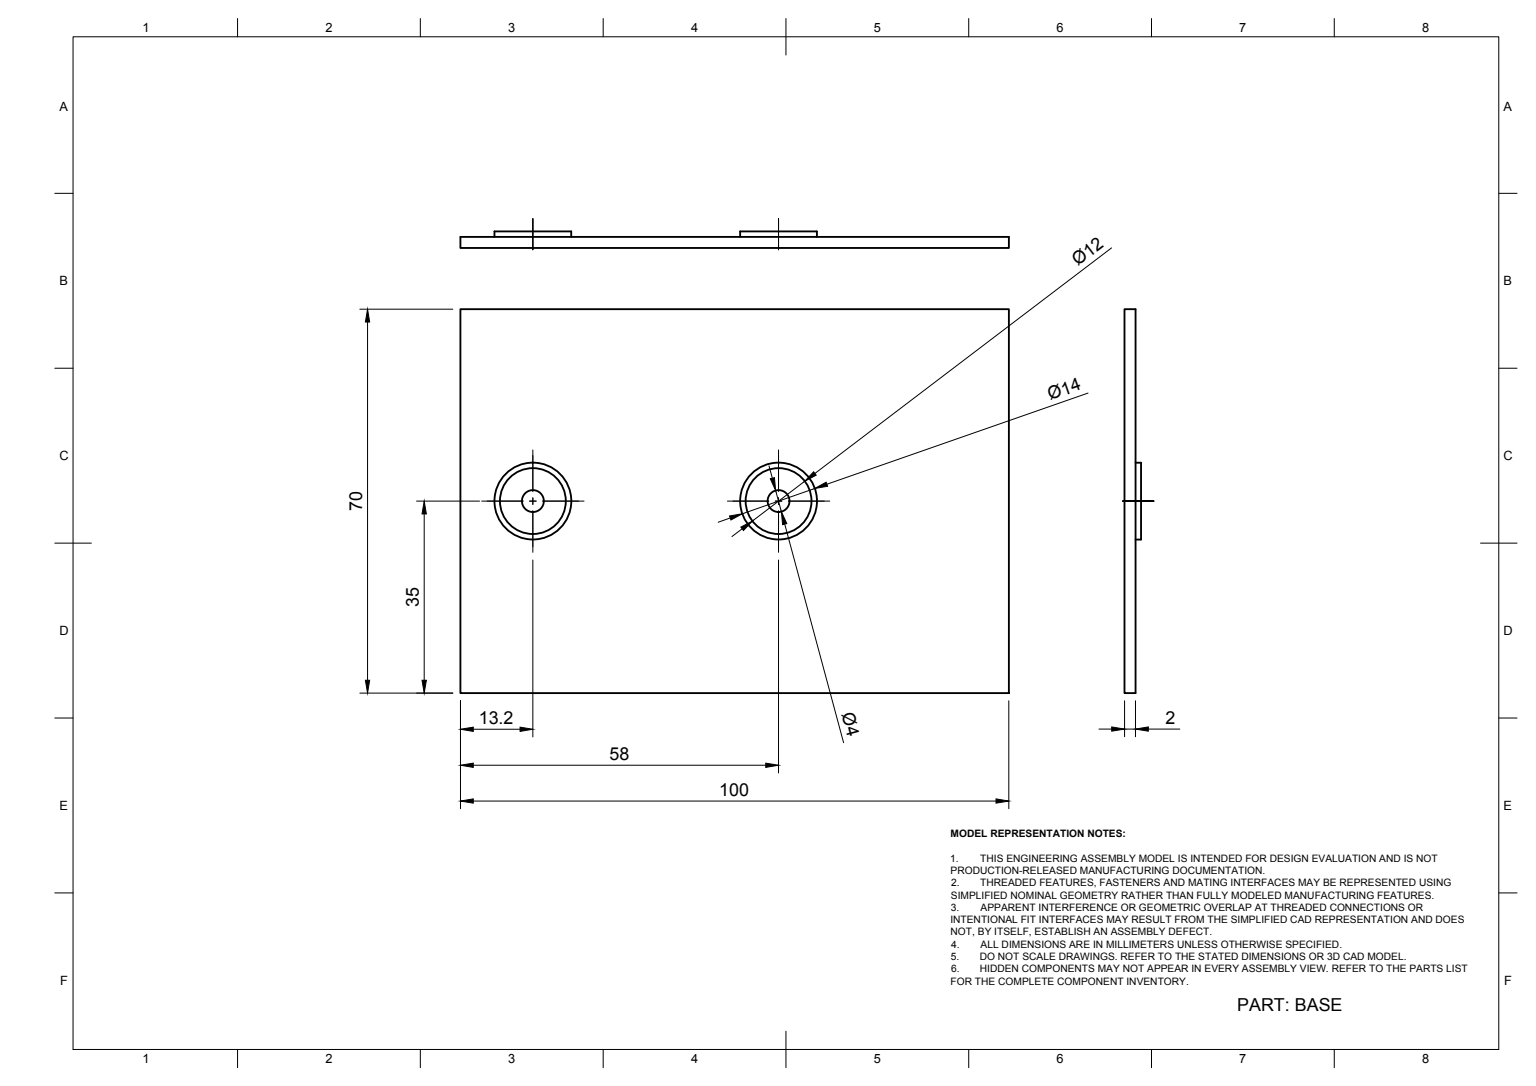
ISO-10303-21;
HEADER;
/* Generated by software containing ST-Developer
 * from STEP Tools, Inc. (www.steptools.com) 
 */

FILE_DESCRIPTION(
/* description */ (''),
/* implementation_level */ '2;1');

FILE_NAME(
/* name */ 'Base.step',
/* time_stamp */ '2026-10-04T15:18:51-07:00',
/* author */ (''),
/* organization */ (''),
/* preprocessor_version */ 'ST-DEVELOPER v20.2',
/* originating_system */ 'Autodesk Translation Framework v15.15.0.0',
/* authorisation */ '');

FILE_SCHEMA (('AUTOMOTIVE_DESIGN { 1 0 10303 214 3 1 1 }'));
ENDSEC;

DATA;
#10=MECHANICAL_DESIGN_GEOMETRIC_PRESENTATION_REPRESENTATION('',(#73),#9891);
#54=SHAPE_REPRESENTATION_RELATIONSHIP('SRR','None',#9925,#62);
#62=ADVANCED_BREP_SHAPE_REPRESENTATION('',(#87),#9885);
#73=STYLED_ITEM('',(#9974),#87);
#87=MANIFOLD_SOLID_BREP('Body1',#5621);
#115=FACE_BOUND('',#834,.T.);
#116=FACE_BOUND('',#836,.T.);
#117=FACE_BOUND('',#837,.T.);
#118=FACE_BOUND('',#841,.T.);
#119=FACE_BOUND('',#843,.T.);
#120=FACE_BOUND('',#849,.T.);
#121=FACE_BOUND('',#850,.T.);
#122=FACE_BOUND('',#852,.T.);
#186=PLANE('',#5903);
#187=PLANE('',#5904);
#188=PLANE('',#5911);
#189=PLANE('',#5912);
#190=PLANE('',#5913);
#191=PLANE('',#5914);
#192=PLANE('',#5915);
#193=PLANE('',#5916);
#194=PLANE('',#5917);
#195=PLANE('',#5918);
#480=FACE_OUTER_BOUND('',#829,.T.);
#481=FACE_OUTER_BOUND('',#830,.T.);
#482=FACE_OUTER_BOUND('',#831,.T.);
#483=FACE_OUTER_BOUND('',#832,.T.);
#484=FACE_OUTER_BOUND('',#833,.T.);
#485=FACE_OUTER_BOUND('',#835,.T.);
#486=FACE_OUTER_BOUND('',#838,.T.);
#487=FACE_OUTER_BOUND('',#839,.T.);
#488=FACE_OUTER_BOUND('',#840,.T.);
#489=FACE_OUTER_BOUND('',#842,.T.);
#490=FACE_OUTER_BOUND('',#844,.T.);
#491=FACE_OUTER_BOUND('',#845,.T.);
#492=FACE_OUTER_BOUND('',#846,.T.);
#493=FACE_OUTER_BOUND('',#847,.T.);
#494=FACE_OUTER_BOUND('',#848,.T.);
#495=FACE_OUTER_BOUND('',#851,.T.);
#829=EDGE_LOOP('',(#3906,#3907,#3908,#3909));
#830=EDGE_LOOP('',(#3910,#3911,#3912,#3913));
#831=EDGE_LOOP('',(#3914,#3915,#3916,#3917));
#832=EDGE_LOOP('',(#3918,#3919,#3920,#3921));
#833=EDGE_LOOP('',(#3922));
#834=EDGE_LOOP('',(#3923));
#835=EDGE_LOOP('',(#3924,#3925,#3926,#3927));
#836=EDGE_LOOP('',(#3928));
#837=EDGE_LOOP('',(#3929));
#838=EDGE_LOOP('',(#3930,#3931,#3932,#3933));
#839=EDGE_LOOP('',(#3934,#3935,#3936,#3937));
#840=EDGE_LOOP('',(#3938));
#841=EDGE_LOOP('',(#3939));
#842=EDGE_LOOP('',(#3940));
#843=EDGE_LOOP('',(#3941));
#844=EDGE_LOOP('',(#3942,#3943,#3944,#3945));
#845=EDGE_LOOP('',(#3946,#3947,#3948,#3949));
#846=EDGE_LOOP('',(#3950,#3951,#3952,#3953));
#847=EDGE_LOOP('',(#3954,#3955,#3956,#3957));
#848=EDGE_LOOP('',(#3958,#3959,#3960,#3961));
#849=EDGE_LOOP('',(#3962));
#850=EDGE_LOOP('',(#3963));
#851=EDGE_LOOP('',(#3964));
#852=EDGE_LOOP('',(#3965));
#1163=LINE('',#8464,#1627);
#1164=LINE('',#8470,#1628);
#1165=LINE('',#8476,#1629);
#1166=LINE('',#8482,#1630);
#1167=LINE('',#8488,#1631);
#1168=LINE('',#8490,#1632);
#1169=LINE('',#8492,#1633);
#1170=LINE('',#8493,#1634);
#1171=LINE('',#8500,#1635);
#1172=LINE('',#8505,#1636);
#1173=LINE('',#8510,#1637);
#1174=LINE('',#8512,#1638);
#1175=LINE('',#8513,#1639);
#1176=LINE('',#8516,#1640);
#1177=LINE('',#8517,#1641);
#1178=LINE('',#8520,#1642);
#1179=LINE('',#8521,#1643);
#1180=LINE('',#8523,#1644);
#1627=VECTOR('',#6750,2.);
#1628=VECTOR('',#6757,2.);
#1629=VECTOR('',#6764,6.00000000000001);
#1630=VECTOR('',#6771,7.00000000000001);
#1631=VECTOR('',#6778,10.);
#1632=VECTOR('',#6779,10.);
#1633=VECTOR('',#6780,10.);
#1634=VECTOR('',#6781,10.);
#1635=VECTOR('',#6788,6.00000000000001);
#1636=VECTOR('',#6795,7.00000000000001);
#1637=VECTOR('',#6802,10.);
#1638=VECTOR('',#6803,10.);
#1639=VECTOR('',#6804,10.);
#1640=VECTOR('',#6807,10.);
#1641=VECTOR('',#6808,10.);
#1642=VECTOR('',#6811,10.);
#1643=VECTOR('',#6812,10.);
#1644=VECTOR('',#6815,10.);
#2155=CIRCLE('',#5892,2.);
#2156=CIRCLE('',#5893,2.);
#2157=CIRCLE('',#5895,2.);
#2158=CIRCLE('',#5896,2.);
#2159=CIRCLE('',#5898,6.00000000000001);
#2160=CIRCLE('',#5899,6.00000000000001);
#2161=CIRCLE('',#5901,7.00000000000001);
#2162=CIRCLE('',#5902,7.00000000000001);
#2163=CIRCLE('',#5905,7.00000000000001);
#2164=CIRCLE('',#5907,6.00000000000001);
#2165=CIRCLE('',#5908,6.00000000000001);
#2166=CIRCLE('',#5910,7.00000000000001);
#2443=VERTEX_POINT('',#8461);
#2444=VERTEX_POINT('',#8463);
#2445=VERTEX_POINT('',#8467);
#2446=VERTEX_POINT('',#8469);
#2447=VERTEX_POINT('',#8473);
#2448=VERTEX_POINT('',#8475);
#2449=VERTEX_POINT('',#8479);
#2450=VERTEX_POINT('',#8481);
#2451=VERTEX_POINT('',#8486);
#2452=VERTEX_POINT('',#8487);
#2453=VERTEX_POINT('',#8489);
#2454=VERTEX_POINT('',#8491);
#2455=VERTEX_POINT('',#8494);
#2456=VERTEX_POINT('',#8497);
#2457=VERTEX_POINT('',#8499);
#2458=VERTEX_POINT('',#8503);
#2459=VERTEX_POINT('',#8509);
#2460=VERTEX_POINT('',#8511);
#2461=VERTEX_POINT('',#8515);
#2462=VERTEX_POINT('',#8519);
#2998=EDGE_CURVE('',#2443,#2443,#2155,.T.);
#2999=EDGE_CURVE('',#2443,#2444,#1163,.T.);
#3000=EDGE_CURVE('',#2444,#2444,#2156,.T.);
#3001=EDGE_CURVE('',#2445,#2445,#2157,.T.);
#3002=EDGE_CURVE('',#2445,#2446,#1164,.T.);
#3003=EDGE_CURVE('',#2446,#2446,#2158,.T.);
#3004=EDGE_CURVE('',#2447,#2447,#2159,.T.);
#3005=EDGE_CURVE('',#2447,#2448,#1165,.T.);
#3006=EDGE_CURVE('',#2448,#2448,#2160,.T.);
#3007=EDGE_CURVE('',#2449,#2449,#2161,.T.);
#3008=EDGE_CURVE('',#2449,#2450,#1166,.T.);
#3009=EDGE_CURVE('',#2450,#2450,#2162,.T.);
#3010=EDGE_CURVE('',#2451,#2452,#1167,.T.);
#3011=EDGE_CURVE('',#2453,#2451,#1168,.T.);
#3012=EDGE_CURVE('',#2454,#2453,#1169,.T.);
#3013=EDGE_CURVE('',#2452,#2454,#1170,.T.);
#3014=EDGE_CURVE('',#2455,#2455,#2163,.T.);
#3015=EDGE_CURVE('',#2456,#2456,#2164,.T.);
#3016=EDGE_CURVE('',#2456,#2457,#1171,.T.);
#3017=EDGE_CURVE('',#2457,#2457,#2165,.T.);
#3018=EDGE_CURVE('',#2458,#2458,#2166,.T.);
#3019=EDGE_CURVE('',#2458,#2455,#1172,.T.);
#3020=EDGE_CURVE('',#2451,#2459,#1173,.T.);
#3021=EDGE_CURVE('',#2460,#2459,#1174,.T.);
#3022=EDGE_CURVE('',#2453,#2460,#1175,.T.);
#3023=EDGE_CURVE('',#2461,#2460,#1176,.T.);
#3024=EDGE_CURVE('',#2454,#2461,#1177,.T.);
#3025=EDGE_CURVE('',#2462,#2461,#1178,.T.);
#3026=EDGE_CURVE('',#2452,#2462,#1179,.T.);
#3027=EDGE_CURVE('',#2459,#2462,#1180,.T.);
#3906=ORIENTED_EDGE('',*,*,#2998,.F.);
#3907=ORIENTED_EDGE('',*,*,#2999,.T.);
#3908=ORIENTED_EDGE('',*,*,#3000,.F.);
#3909=ORIENTED_EDGE('',*,*,#2999,.F.);
#3910=ORIENTED_EDGE('',*,*,#3001,.F.);
#3911=ORIENTED_EDGE('',*,*,#3002,.T.);
#3912=ORIENTED_EDGE('',*,*,#3003,.F.);
#3913=ORIENTED_EDGE('',*,*,#3002,.F.);
#3914=ORIENTED_EDGE('',*,*,#3004,.F.);
#3915=ORIENTED_EDGE('',*,*,#3005,.T.);
#3916=ORIENTED_EDGE('',*,*,#3006,.F.);
#3917=ORIENTED_EDGE('',*,*,#3005,.F.);
#3918=ORIENTED_EDGE('',*,*,#3007,.F.);
#3919=ORIENTED_EDGE('',*,*,#3008,.T.);
#3920=ORIENTED_EDGE('',*,*,#3009,.F.);
#3921=ORIENTED_EDGE('',*,*,#3008,.F.);
#3922=ORIENTED_EDGE('',*,*,#3007,.T.);
#3923=ORIENTED_EDGE('',*,*,#3006,.T.);
#3924=ORIENTED_EDGE('',*,*,#3010,.F.);
#3925=ORIENTED_EDGE('',*,*,#3011,.F.);
#3926=ORIENTED_EDGE('',*,*,#3012,.F.);
#3927=ORIENTED_EDGE('',*,*,#3013,.F.);
#3928=ORIENTED_EDGE('',*,*,#3014,.T.);
#3929=ORIENTED_EDGE('',*,*,#3009,.T.);
#3930=ORIENTED_EDGE('',*,*,#3015,.F.);
#3931=ORIENTED_EDGE('',*,*,#3016,.T.);
#3932=ORIENTED_EDGE('',*,*,#3017,.F.);
#3933=ORIENTED_EDGE('',*,*,#3016,.F.);
#3934=ORIENTED_EDGE('',*,*,#3018,.F.);
#3935=ORIENTED_EDGE('',*,*,#3019,.T.);
#3936=ORIENTED_EDGE('',*,*,#3014,.F.);
#3937=ORIENTED_EDGE('',*,*,#3019,.F.);
#3938=ORIENTED_EDGE('',*,*,#3018,.T.);
#3939=ORIENTED_EDGE('',*,*,#3017,.T.);
#3940=ORIENTED_EDGE('',*,*,#3004,.T.);
#3941=ORIENTED_EDGE('',*,*,#3001,.T.);
#3942=ORIENTED_EDGE('',*,*,#3011,.T.);
#3943=ORIENTED_EDGE('',*,*,#3020,.T.);
#3944=ORIENTED_EDGE('',*,*,#3021,.F.);
#3945=ORIENTED_EDGE('',*,*,#3022,.F.);
#3946=ORIENTED_EDGE('',*,*,#3012,.T.);
#3947=ORIENTED_EDGE('',*,*,#3022,.T.);
#3948=ORIENTED_EDGE('',*,*,#3023,.F.);
#3949=ORIENTED_EDGE('',*,*,#3024,.F.);
#3950=ORIENTED_EDGE('',*,*,#3013,.T.);
#3951=ORIENTED_EDGE('',*,*,#3024,.T.);
#3952=ORIENTED_EDGE('',*,*,#3025,.F.);
#3953=ORIENTED_EDGE('',*,*,#3026,.F.);
#3954=ORIENTED_EDGE('',*,*,#3010,.T.);
#3955=ORIENTED_EDGE('',*,*,#3026,.T.);
#3956=ORIENTED_EDGE('',*,*,#3027,.F.);
#3957=ORIENTED_EDGE('',*,*,#3020,.F.);
#3958=ORIENTED_EDGE('',*,*,#3027,.T.);
#3959=ORIENTED_EDGE('',*,*,#3025,.T.);
#3960=ORIENTED_EDGE('',*,*,#3023,.T.);
#3961=ORIENTED_EDGE('',*,*,#3021,.T.);
#3962=ORIENTED_EDGE('',*,*,#3000,.T.);
#3963=ORIENTED_EDGE('',*,*,#3003,.T.);
#3964=ORIENTED_EDGE('',*,*,#3015,.T.);
#3965=ORIENTED_EDGE('',*,*,#2998,.T.);
#5214=CYLINDRICAL_SURFACE('',#5891,2.);
#5215=CYLINDRICAL_SURFACE('',#5894,2.);
#5216=CYLINDRICAL_SURFACE('',#5897,6.00000000000001);
#5217=CYLINDRICAL_SURFACE('',#5900,7.00000000000001);
#5218=CYLINDRICAL_SURFACE('',#5906,6.00000000000001);
#5219=CYLINDRICAL_SURFACE('',#5909,7.00000000000001);
#5359=ADVANCED_FACE('',(#480),#5214,.F.);
#5360=ADVANCED_FACE('',(#481),#5215,.F.);
#5361=ADVANCED_FACE('',(#482),#5216,.F.);
#5362=ADVANCED_FACE('',(#483),#5217,.T.);
#5363=ADVANCED_FACE('',(#484,#115),#186,.T.);
#5364=ADVANCED_FACE('',(#485,#116,#117),#187,.F.);
#5365=ADVANCED_FACE('',(#486),#5218,.F.);
#5366=ADVANCED_FACE('',(#487),#5219,.T.);
#5367=ADVANCED_FACE('',(#488,#118),#188,.T.);
#5368=ADVANCED_FACE('',(#489,#119),#189,.F.);
#5369=ADVANCED_FACE('',(#490),#190,.T.);
#5370=ADVANCED_FACE('',(#491),#191,.T.);
#5371=ADVANCED_FACE('',(#492),#192,.T.);
#5372=ADVANCED_FACE('',(#493),#193,.T.);
#5373=ADVANCED_FACE('',(#494,#120,#121),#194,.T.);
#5374=ADVANCED_FACE('',(#495,#122),#195,.F.);
#5621=CLOSED_SHELL('',(#5359,#5360,#5361,#5362,#5363,#5364,#5365,#5366,
#5367,#5368,#5369,#5370,#5371,#5372,#5373,#5374));
#5890=AXIS2_PLACEMENT_3D('',#8459,#6744,#6745);
#5891=AXIS2_PLACEMENT_3D('',#8460,#6746,#6747);
#5892=AXIS2_PLACEMENT_3D('',#8462,#6748,#6749);
#5893=AXIS2_PLACEMENT_3D('',#8465,#6751,#6752);
#5894=AXIS2_PLACEMENT_3D('',#8466,#6753,#6754);
#5895=AXIS2_PLACEMENT_3D('',#8468,#6755,#6756);
#5896=AXIS2_PLACEMENT_3D('',#8471,#6758,#6759);
#5897=AXIS2_PLACEMENT_3D('',#8472,#6760,#6761);
#5898=AXIS2_PLACEMENT_3D('',#8474,#6762,#6763);
#5899=AXIS2_PLACEMENT_3D('',#8477,#6765,#6766);
#5900=AXIS2_PLACEMENT_3D('',#8478,#6767,#6768);
#5901=AXIS2_PLACEMENT_3D('',#8480,#6769,#6770);
#5902=AXIS2_PLACEMENT_3D('',#8483,#6772,#6773);
#5903=AXIS2_PLACEMENT_3D('',#8484,#6774,#6775);
#5904=AXIS2_PLACEMENT_3D('',#8485,#6776,#6777);
#5905=AXIS2_PLACEMENT_3D('',#8495,#6782,#6783);
#5906=AXIS2_PLACEMENT_3D('',#8496,#6784,#6785);
#5907=AXIS2_PLACEMENT_3D('',#8498,#6786,#6787);
#5908=AXIS2_PLACEMENT_3D('',#8501,#6789,#6790);
#5909=AXIS2_PLACEMENT_3D('',#8502,#6791,#6792);
#5910=AXIS2_PLACEMENT_3D('',#8504,#6793,#6794);
#5911=AXIS2_PLACEMENT_3D('',#8506,#6796,#6797);
#5912=AXIS2_PLACEMENT_3D('',#8507,#6798,#6799);
#5913=AXIS2_PLACEMENT_3D('',#8508,#6800,#6801);
#5914=AXIS2_PLACEMENT_3D('',#8514,#6805,#6806);
#5915=AXIS2_PLACEMENT_3D('',#8518,#6809,#6810);
#5916=AXIS2_PLACEMENT_3D('',#8522,#6813,#6814);
#5917=AXIS2_PLACEMENT_3D('',#8524,#6816,#6817);
#5918=AXIS2_PLACEMENT_3D('',#8525,#6818,#6819);
#6744=DIRECTION('axis',(0.,0.,1.));
#6745=DIRECTION('refdir',(1.,0.,0.));
#6746=DIRECTION('center_axis',(0.,1.,0.));
#6747=DIRECTION('ref_axis',(1.,0.,0.));
#6748=DIRECTION('center_axis',(0.,1.,0.));
#6749=DIRECTION('ref_axis',(1.,0.,0.));
#6750=DIRECTION('',(0.,1.,0.));
#6751=DIRECTION('center_axis',(0.,-1.,0.));
#6752=DIRECTION('ref_axis',(1.,0.,0.));
#6753=DIRECTION('center_axis',(0.,1.,0.));
#6754=DIRECTION('ref_axis',(1.,0.,0.));
#6755=DIRECTION('center_axis',(0.,1.,0.));
#6756=DIRECTION('ref_axis',(1.,0.,0.));
#6757=DIRECTION('',(0.,1.,0.));
#6758=DIRECTION('center_axis',(0.,-1.,0.));
#6759=DIRECTION('ref_axis',(1.,0.,0.));
#6760=DIRECTION('center_axis',(0.,-1.,0.));
#6761=DIRECTION('ref_axis',(1.,0.,0.));
#6762=DIRECTION('center_axis',(0.,-1.,0.));
#6763=DIRECTION('ref_axis',(1.,0.,0.));
#6764=DIRECTION('',(0.,-1.,0.));
#6765=DIRECTION('center_axis',(0.,1.,0.));
#6766=DIRECTION('ref_axis',(1.,0.,0.));
#6767=DIRECTION('center_axis',(0.,-1.,0.));
#6768=DIRECTION('ref_axis',(1.,0.,0.));
#6769=DIRECTION('center_axis',(0.,-1.,0.));
#6770=DIRECTION('ref_axis',(1.,0.,0.));
#6771=DIRECTION('',(0.,1.,0.));
#6772=DIRECTION('center_axis',(0.,1.,0.));
#6773=DIRECTION('ref_axis',(1.,0.,0.));
#6774=DIRECTION('center_axis',(0.,-1.,0.));
#6775=DIRECTION('ref_axis',(1.,0.,0.));
#6776=DIRECTION('center_axis',(0.,1.,0.));
#6777=DIRECTION('ref_axis',(1.,0.,0.));
#6778=DIRECTION('',(0.,0.,-1.));
#6779=DIRECTION('',(1.,0.,0.));
#6780=DIRECTION('',(0.,0.,1.));
#6781=DIRECTION('',(-1.,0.,0.));
#6782=DIRECTION('center_axis',(0.,1.,0.));
#6783=DIRECTION('ref_axis',(1.,0.,0.));
#6784=DIRECTION('center_axis',(0.,-1.,0.));
#6785=DIRECTION('ref_axis',(1.,0.,0.));
#6786=DIRECTION('center_axis',(0.,-1.,0.));
#6787=DIRECTION('ref_axis',(1.,0.,0.));
#6788=DIRECTION('',(0.,-1.,0.));
#6789=DIRECTION('center_axis',(0.,1.,0.));
#6790=DIRECTION('ref_axis',(1.,0.,0.));
#6791=DIRECTION('center_axis',(0.,-1.,0.));
#6792=DIRECTION('ref_axis',(1.,0.,0.));
#6793=DIRECTION('center_axis',(0.,-1.,0.));
#6794=DIRECTION('ref_axis',(1.,0.,0.));
#6795=DIRECTION('',(0.,1.,0.));
#6796=DIRECTION('center_axis',(0.,-1.,0.));
#6797=DIRECTION('ref_axis',(1.,0.,0.));
#6798=DIRECTION('center_axis',(0.,1.,0.));
#6799=DIRECTION('ref_axis',(1.,0.,0.));
#6800=DIRECTION('center_axis',(0.,0.,1.));
#6801=DIRECTION('ref_axis',(1.,0.,0.));
#6802=DIRECTION('',(0.,1.,0.));
#6803=DIRECTION('',(1.,0.,0.));
#6804=DIRECTION('',(0.,1.,0.));
#6805=DIRECTION('center_axis',(-1.,0.,0.));
#6806=DIRECTION('ref_axis',(0.,0.,1.));
#6807=DIRECTION('',(0.,0.,1.));
#6808=DIRECTION('',(0.,1.,0.));
#6809=DIRECTION('center_axis',(0.,0.,-1.));
#6810=DIRECTION('ref_axis',(-1.,0.,0.));
#6811=DIRECTION('',(-1.,0.,0.));
#6812=DIRECTION('',(0.,1.,0.));
#6813=DIRECTION('center_axis',(1.,0.,0.));
#6814=DIRECTION('ref_axis',(0.,0.,-1.));
#6815=DIRECTION('',(0.,0.,-1.));
#6816=DIRECTION('center_axis',(0.,1.,0.));
#6817=DIRECTION('ref_axis',(0.,0.,1.));
#6818=DIRECTION('center_axis',(0.,1.,0.));
#6819=DIRECTION('ref_axis',(1.,0.,0.));
#8459=CARTESIAN_POINT('',(0.,0.,0.));
#8460=CARTESIAN_POINT('Origin',(3.44895709521403E-16,0.,86.8));
#8461=CARTESIAN_POINT('',(-2.,0.,86.8));
#8462=CARTESIAN_POINT('Origin',(3.44895709521403E-16,0.,86.8));
#8463=CARTESIAN_POINT('',(-2.,2.,86.8));
#8464=CARTESIAN_POINT('',(-2.,0.,86.8));
#8465=CARTESIAN_POINT('Origin',(3.44895709521403E-16,2.,86.8));
#8466=CARTESIAN_POINT('Origin',(5.11429163215176E-16,0.,42.));
#8467=CARTESIAN_POINT('',(-2.,0.,42.));
#8468=CARTESIAN_POINT('Origin',(5.11429163215176E-16,0.,42.));
#8469=CARTESIAN_POINT('',(-2.,2.,42.));
#8470=CARTESIAN_POINT('',(-2.,0.,42.));
#8471=CARTESIAN_POINT('Origin',(5.11429163215176E-16,2.,42.));
#8472=CARTESIAN_POINT('Origin',(5.11429163215176E-16,0.,42.));
#8473=CARTESIAN_POINT('',(-6.00000000000001,0.,42.));
#8474=CARTESIAN_POINT('Origin',(5.11429163215176E-16,0.,42.));
#8475=CARTESIAN_POINT('',(-6.00000000000001,-1.,42.));
#8476=CARTESIAN_POINT('',(-6.00000000000001,0.,42.));
#8477=CARTESIAN_POINT('Origin',(5.11429163215176E-16,-1.,42.));
#8478=CARTESIAN_POINT('Origin',(5.11429163215176E-16,0.,42.));
#8479=CARTESIAN_POINT('',(-7.00000000000001,-1.,42.));
#8480=CARTESIAN_POINT('Origin',(5.11429163215176E-16,-1.,42.));
#8481=CARTESIAN_POINT('',(-7.00000000000001,0.,42.));
#8482=CARTESIAN_POINT('',(-7.00000000000001,0.,42.));
#8483=CARTESIAN_POINT('Origin',(5.11429163215176E-16,0.,42.));
#8484=CARTESIAN_POINT('Origin',(0.,-1.,42.));
#8485=CARTESIAN_POINT('Origin',(0.,0.,50.));
#8486=CARTESIAN_POINT('',(35.,0.,100.));
#8487=CARTESIAN_POINT('',(35.,0.,0.));
#8488=CARTESIAN_POINT('',(35.,0.,100.));
#8489=CARTESIAN_POINT('',(-35.,0.,100.));
#8490=CARTESIAN_POINT('',(-35.,0.,100.));
#8491=CARTESIAN_POINT('',(-35.,0.,0.));
#8492=CARTESIAN_POINT('',(-35.,0.,0.));
#8493=CARTESIAN_POINT('',(35.,0.,0.));
#8494=CARTESIAN_POINT('',(-7.00000000000001,0.,86.8));
#8495=CARTESIAN_POINT('Origin',(5.11429163215176E-16,0.,86.8));
#8496=CARTESIAN_POINT('Origin',(5.11429163215176E-16,0.,86.8));
#8497=CARTESIAN_POINT('',(-6.00000000000001,0.,86.8));
#8498=CARTESIAN_POINT('Origin',(5.11429163215176E-16,0.,86.8));
#8499=CARTESIAN_POINT('',(-6.00000000000001,-1.,86.8));
#8500=CARTESIAN_POINT('',(-6.00000000000001,0.,86.8));
#8501=CARTESIAN_POINT('Origin',(5.11429163215176E-16,-1.,86.8));
#8502=CARTESIAN_POINT('Origin',(5.11429163215176E-16,0.,86.8));
#8503=CARTESIAN_POINT('',(-7.00000000000001,-1.,86.8));
#8504=CARTESIAN_POINT('Origin',(5.11429163215176E-16,-1.,86.8));
#8505=CARTESIAN_POINT('',(-7.00000000000001,0.,86.8));
#8506=CARTESIAN_POINT('Origin',(0.,-1.,86.8));
#8507=CARTESIAN_POINT('Origin',(0.,0.,50.));
#8508=CARTESIAN_POINT('Origin',(-35.,0.,100.));
#8509=CARTESIAN_POINT('',(35.,2.,100.));
#8510=CARTESIAN_POINT('',(35.,0.,100.));
#8511=CARTESIAN_POINT('',(-35.,2.,100.));
#8512=CARTESIAN_POINT('',(-35.,2.,100.));
#8513=CARTESIAN_POINT('',(-35.,0.,100.));
#8514=CARTESIAN_POINT('Origin',(-35.,0.,0.));
#8515=CARTESIAN_POINT('',(-35.,2.,0.));
#8516=CARTESIAN_POINT('',(-35.,2.,0.));
#8517=CARTESIAN_POINT('',(-35.,0.,0.));
#8518=CARTESIAN_POINT('Origin',(35.,0.,0.));
#8519=CARTESIAN_POINT('',(35.,2.,0.));
#8520=CARTESIAN_POINT('',(35.,2.,0.));
#8521=CARTESIAN_POINT('',(35.,0.,0.));
#8522=CARTESIAN_POINT('Origin',(35.,0.,100.));
#8523=CARTESIAN_POINT('',(35.,2.,100.));
#8524=CARTESIAN_POINT('Origin',(0.,2.,50.));
#8525=CARTESIAN_POINT('Origin',(0.,0.,50.));
#9875=UNCERTAINTY_MEASURE_WITH_UNIT(LENGTH_MEASURE(0.01),#9892,
'DISTANCE_ACCURACY_VALUE',
'Maximum model space distance between geometric entities at asserted c
onnectivities');
#9881=UNCERTAINTY_MEASURE_WITH_UNIT(LENGTH_MEASURE(0.01),#9892,
'DISTANCE_ACCURACY_VALUE',
'Maximum model space distance between geometric entities at asserted c
onnectivities');
#9885=(
GEOMETRIC_REPRESENTATION_CONTEXT(3)
GLOBAL_UNCERTAINTY_ASSIGNED_CONTEXT((#9875))
GLOBAL_UNIT_ASSIGNED_CONTEXT((#9892,#9894,#9895))
REPRESENTATION_CONTEXT('','3D')
);
#9891=(
GEOMETRIC_REPRESENTATION_CONTEXT(3)
GLOBAL_UNCERTAINTY_ASSIGNED_CONTEXT((#9881))
GLOBAL_UNIT_ASSIGNED_CONTEXT((#9892,#9894,#9895))
REPRESENTATION_CONTEXT('','3D')
);
#9892=(
LENGTH_UNIT()
NAMED_UNIT(*)
SI_UNIT(.MILLI.,.METRE.)
);
#9894=(
NAMED_UNIT(*)
PLANE_ANGLE_UNIT()
SI_UNIT($,.RADIAN.)
);
#9895=(
NAMED_UNIT(*)
SI_UNIT($,.STERADIAN.)
SOLID_ANGLE_UNIT()
);
#9899=SHAPE_DEFINITION_REPRESENTATION(#9908,#9925);
#9908=PRODUCT_DEFINITION_SHAPE('',$,#9935);
#9925=SHAPE_REPRESENTATION('',(#5890),#9885);
#9931=PRODUCT_DEFINITION_CONTEXT('part definition',#9960,'design');
#9935=PRODUCT_DEFINITION('base','Base',#9944,#9931);
#9944=PRODUCT_DEFINITION_FORMATION('',$,#9965);
#9960=APPLICATION_CONTEXT(
'Core Data for Automotive Mechanical Design Process');
#9961=PRODUCT_CONTEXT('part definition',#9960,'mechanical');
#9965=PRODUCT('base','Base',$,(#9961));
#9974=PRESENTATION_STYLE_ASSIGNMENT((#9979));
#9979=SURFACE_STYLE_USAGE(.BOTH.,#9984);
#9984=SURFACE_SIDE_STYLE('',(#9989));
#9989=SURFACE_STYLE_FILL_AREA(#9994);
#9994=FILL_AREA_STYLE('Opaque(255,242,183)',(#9999));
#9999=FILL_AREA_STYLE_COLOUR('Opaque(255,242,183)',#10004);
#10004=COLOUR_RGB('Opaque(255,242,183)', 0.08235294, 0.09019608, 0.10196078);
ENDSEC;
END-ISO-10303-21;
